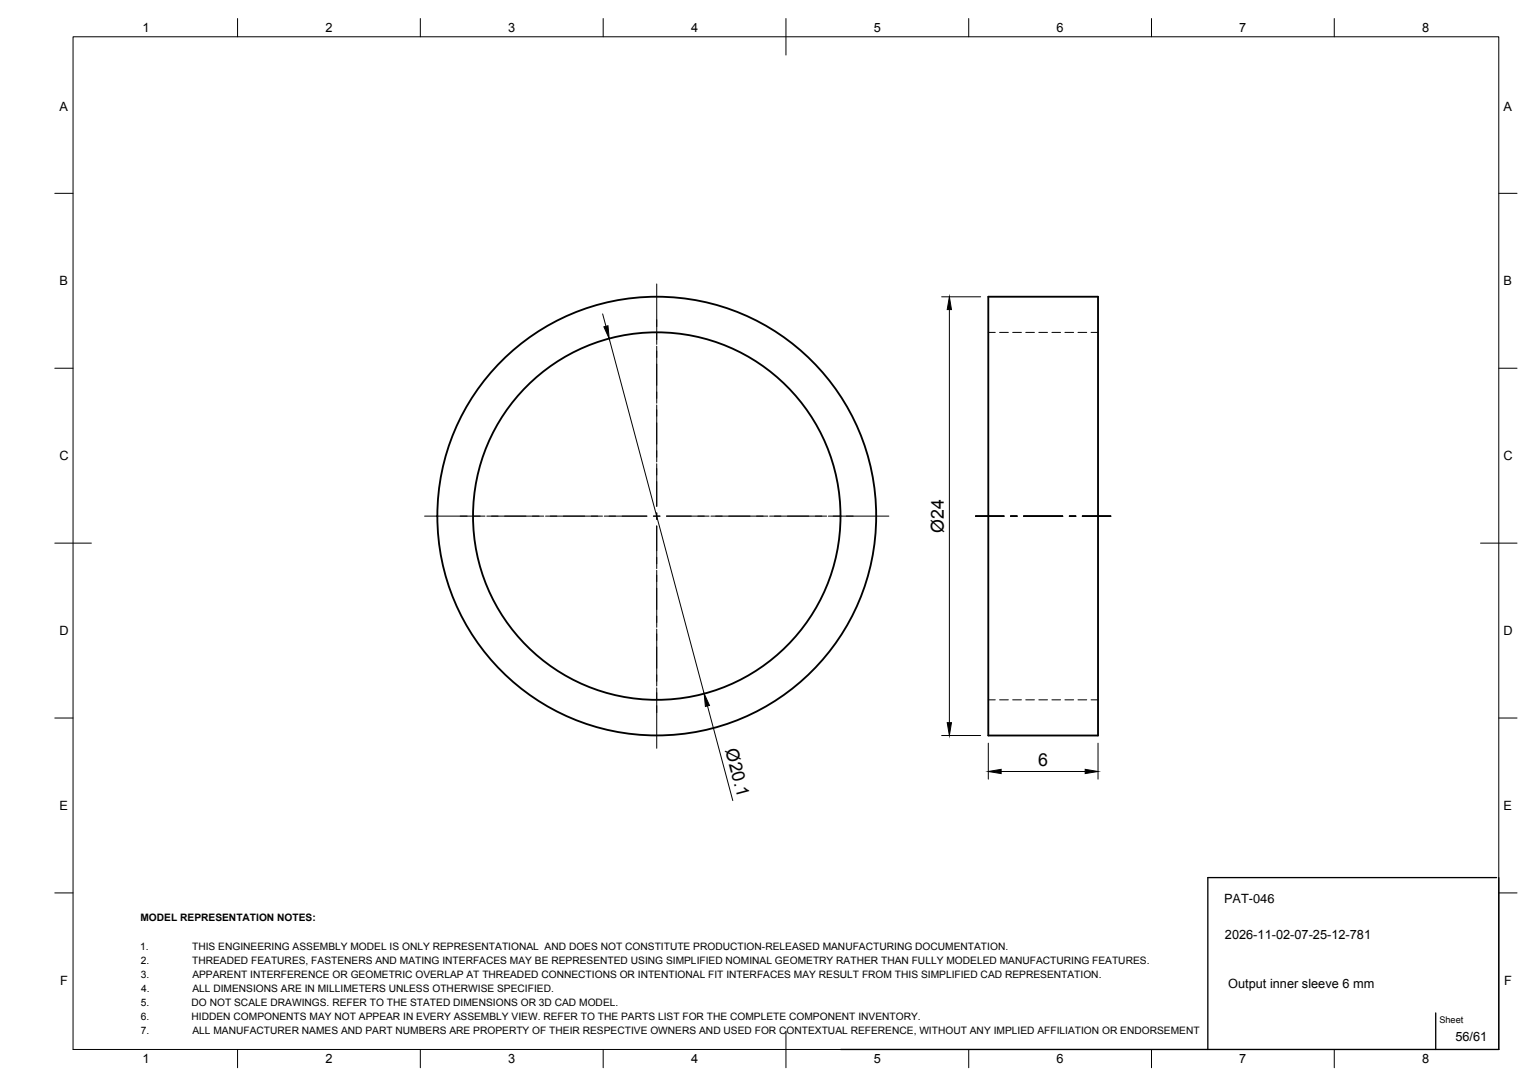
ISO-10303-21;
HEADER;
/* Generated by software containing ST-Developer
 * from STEP Tools, Inc. (www.steptools.com) 
 */

FILE_DESCRIPTION(
/* description */ ('Gear mesh backlash fixture'),
/* implementation_level */ '2;1');

FILE_NAME(
/* name */ 'Output inner sleeve 6 mm.step',
/* time_stamp */ '2026-10-28T03:26:00-07:00',
/* author */ (''),
/* organization */ (''),
/* preprocessor_version */ 'ST-DEVELOPER v20.2',
/* originating_system */ 'Autodesk Translation Framework v15.17.0.0',
/* authorisation */ '');

FILE_SCHEMA (('AUTOMOTIVE_DESIGN { 1 0 10303 214 3 1 1 }'));
ENDSEC;

DATA;
#10=MECHANICAL_DESIGN_GEOMETRIC_PRESENTATION_REPRESENTATION('',(#1073),#57900);
#958=SHAPE_REPRESENTATION_RELATIONSHIP('SRR','None',#58159,#1008);
#1008=ADVANCED_BREP_SHAPE_REPRESENTATION('',(#1136),#57892);
#1073=STYLED_ITEM('',(#58479),#1136);
#1136=MANIFOLD_SOLID_BREP('Body1',#13635);
#1315=FACE_BOUND('',#3181,.T.);
#1316=FACE_BOUND('',#3183,.T.);
#1614=PLANE('',#15254);
#1615=PLANE('',#15255);
#2241=FACE_OUTER_BOUND('',#3178,.T.);
#2242=FACE_OUTER_BOUND('',#3179,.T.);
#2243=FACE_OUTER_BOUND('',#3180,.T.);
#2244=FACE_OUTER_BOUND('',#3182,.T.);
#3178=EDGE_LOOP('',(#11407,#11408,#11409,#11410));
#3179=EDGE_LOOP('',(#11411,#11412,#11413,#11414));
#3180=EDGE_LOOP('',(#11415));
#3181=EDGE_LOOP('',(#11416));
#3182=EDGE_LOOP('',(#11417));
#3183=EDGE_LOOP('',(#11418));
#4065=LINE('',#33878,#4954);
#4066=LINE('',#33884,#4955);
#4954=VECTOR('',#18342,1.005);
#4955=VECTOR('',#18349,1.2);
#5671=CIRCLE('',#15249,1.005);
#5672=CIRCLE('',#15250,1.005);
#5673=CIRCLE('',#15252,1.2);
#5674=CIRCLE('',#15253,1.2);
#6634=VERTEX_POINT('',#33875);
#6635=VERTEX_POINT('',#33877);
#6636=VERTEX_POINT('',#33881);
#6637=VERTEX_POINT('',#33883);
#8290=EDGE_CURVE('',#6634,#6634,#5671,.T.);
#8291=EDGE_CURVE('',#6634,#6635,#4065,.T.);
#8292=EDGE_CURVE('',#6635,#6635,#5672,.T.);
#8293=EDGE_CURVE('',#6636,#6636,#5673,.T.);
#8294=EDGE_CURVE('',#6636,#6637,#4066,.T.);
#8295=EDGE_CURVE('',#6637,#6637,#5674,.T.);
#11407=ORIENTED_EDGE('',*,*,#8290,.F.);
#11408=ORIENTED_EDGE('',*,*,#8291,.T.);
#11409=ORIENTED_EDGE('',*,*,#8292,.T.);
#11410=ORIENTED_EDGE('',*,*,#8291,.F.);
#11411=ORIENTED_EDGE('',*,*,#8293,.F.);
#11412=ORIENTED_EDGE('',*,*,#8294,.T.);
#11413=ORIENTED_EDGE('',*,*,#8295,.T.);
#11414=ORIENTED_EDGE('',*,*,#8294,.F.);
#11415=ORIENTED_EDGE('',*,*,#8293,.T.);
#11416=ORIENTED_EDGE('',*,*,#8290,.T.);
#11417=ORIENTED_EDGE('',*,*,#8295,.F.);
#11418=ORIENTED_EDGE('',*,*,#8292,.F.);
#12757=CYLINDRICAL_SURFACE('',#15248,1.005);
#12758=CYLINDRICAL_SURFACE('',#15251,1.2);
#13358=ADVANCED_FACE('',(#2241),#12757,.F.);
#13359=ADVANCED_FACE('',(#2242),#12758,.T.);
#13360=ADVANCED_FACE('',(#2243,#1315),#1614,.T.);
#13361=ADVANCED_FACE('',(#2244,#1316),#1615,.F.);
#13635=CLOSED_SHELL('',(#13358,#13359,#13360,#13361));
#15247=AXIS2_PLACEMENT_3D('',#33873,#18336,#18337);
#15248=AXIS2_PLACEMENT_3D('',#33874,#18338,#18339);
#15249=AXIS2_PLACEMENT_3D('',#33876,#18340,#18341);
#15250=AXIS2_PLACEMENT_3D('',#33879,#18343,#18344);
#15251=AXIS2_PLACEMENT_3D('',#33880,#18345,#18346);
#15252=AXIS2_PLACEMENT_3D('',#33882,#18347,#18348);
#15253=AXIS2_PLACEMENT_3D('',#33885,#18350,#18351);
#15254=AXIS2_PLACEMENT_3D('',#33886,#18352,#18353);
#15255=AXIS2_PLACEMENT_3D('',#33887,#18354,#18355);
#18336=DIRECTION('axis',(0.,0.,1.));
#18337=DIRECTION('refdir',(1.,0.,0.));
#18338=DIRECTION('center_axis',(0.,0.,1.));
#18339=DIRECTION('ref_axis',(1.,0.,0.));
#18340=DIRECTION('center_axis',(0.,0.,-1.));
#18341=DIRECTION('ref_axis',(1.,0.,0.));
#18342=DIRECTION('',(0.,0.,-1.));
#18343=DIRECTION('center_axis',(0.,0.,-1.));
#18344=DIRECTION('ref_axis',(1.,0.,0.));
#18345=DIRECTION('center_axis',(0.,0.,1.));
#18346=DIRECTION('ref_axis',(1.,0.,0.));
#18347=DIRECTION('center_axis',(0.,0.,1.));
#18348=DIRECTION('ref_axis',(1.,0.,0.));
#18349=DIRECTION('',(0.,0.,-1.));
#18350=DIRECTION('center_axis',(0.,0.,1.));
#18351=DIRECTION('ref_axis',(1.,0.,0.));
#18352=DIRECTION('center_axis',(0.,0.,1.));
#18353=DIRECTION('ref_axis',(1.,0.,0.));
#18354=DIRECTION('center_axis',(0.,0.,1.));
#18355=DIRECTION('ref_axis',(1.,0.,0.));
#33873=CARTESIAN_POINT('',(0.,0.,0.));
#33874=CARTESIAN_POINT('Origin',(6.,0.,7.2));
#33875=CARTESIAN_POINT('',(4.995,-1.23077003314309E-16,7.8));
#33876=CARTESIAN_POINT('Origin',(6.,0.,7.8));
#33877=CARTESIAN_POINT('',(4.995,-1.23077003314309E-16,7.2));
#33878=CARTESIAN_POINT('',(4.995,-1.23077003314309E-16,7.2));
#33879=CARTESIAN_POINT('Origin',(6.,0.,7.2));
#33880=CARTESIAN_POINT('Origin',(6.,0.,7.2));
#33881=CARTESIAN_POINT('',(4.8,-1.46957615897682E-16,7.8));
#33882=CARTESIAN_POINT('Origin',(6.,0.,7.8));
#33883=CARTESIAN_POINT('',(4.8,-1.46957615897682E-16,7.2));
#33884=CARTESIAN_POINT('',(4.8,-1.46957615897682E-16,7.2));
#33885=CARTESIAN_POINT('Origin',(6.,0.,7.2));
#33886=CARTESIAN_POINT('Origin',(6.,0.,7.8));
#33887=CARTESIAN_POINT('Origin',(6.,0.,7.2));
#57833=UNCERTAINTY_MEASURE_WITH_UNIT(LENGTH_MEASURE(0.001),#57901,
'DISTANCE_ACCURACY_VALUE',
'Maximum model space distance between geometric entities at asserted c
onnectivities');
#57841=UNCERTAINTY_MEASURE_WITH_UNIT(LENGTH_MEASURE(0.001),#57901,
'DISTANCE_ACCURACY_VALUE',
'Maximum model space distance between geometric entities at asserted c
onnectivities');
#57892=(
GEOMETRIC_REPRESENTATION_CONTEXT(3)
GLOBAL_UNCERTAINTY_ASSIGNED_CONTEXT((#57833))
GLOBAL_UNIT_ASSIGNED_CONTEXT((#57901,#57903,#57904))
REPRESENTATION_CONTEXT('','3D')
);
#57900=(
GEOMETRIC_REPRESENTATION_CONTEXT(3)
GLOBAL_UNCERTAINTY_ASSIGNED_CONTEXT((#57841))
GLOBAL_UNIT_ASSIGNED_CONTEXT((#57901,#57903,#57904))
REPRESENTATION_CONTEXT('','3D')
);
#57901=(
LENGTH_UNIT()
NAMED_UNIT(*)
SI_UNIT(.CENTI.,.METRE.)
);
#57903=(
NAMED_UNIT(*)
PLANE_ANGLE_UNIT()
SI_UNIT($,.RADIAN.)
);
#57904=(
NAMED_UNIT(*)
SI_UNIT($,.STERADIAN.)
SOLID_ANGLE_UNIT()
);
#57955=SHAPE_DEFINITION_REPRESENTATION(#58026,#58159);
#58026=PRODUCT_DEFINITION_SHAPE('',$,#58218);
#58159=SHAPE_REPRESENTATION('',(#15247),#57892);
#58167=PRODUCT_DEFINITION_CONTEXT('part definition',#58343,'design');
#58218=PRODUCT_DEFINITION('Output inner sleeve 6 mm',
'Output inner sleeve 6 mm',#58276,#58167);
#58276=PRODUCT_DEFINITION_FORMATION('',$,#58395);
#58343=APPLICATION_CONTEXT(
'Core Data for Automotive Mechanical Design Process');
#58344=PRODUCT_CONTEXT('part definition',#58343,'mechanical');
#58395=PRODUCT('Output inner sleeve 6 mm','Output inner sleeve 6 mm',
'Output inner sleeve 6 mm',(#58344));
#58473=COLOUR_RGB('Off White',0.89,0.88,0.83);
#58474=FILL_AREA_STYLE_COLOUR('',#58473);
#58475=FILL_AREA_STYLE('',(#58474));
#58476=SURFACE_STYLE_FILL_AREA(#58475);
#58477=SURFACE_SIDE_STYLE('',(#58476));
#58478=SURFACE_STYLE_USAGE(.BOTH.,#58477);
#58479=PRESENTATION_STYLE_ASSIGNMENT((#58478));
ENDSEC;
END-ISO-10303-21;
